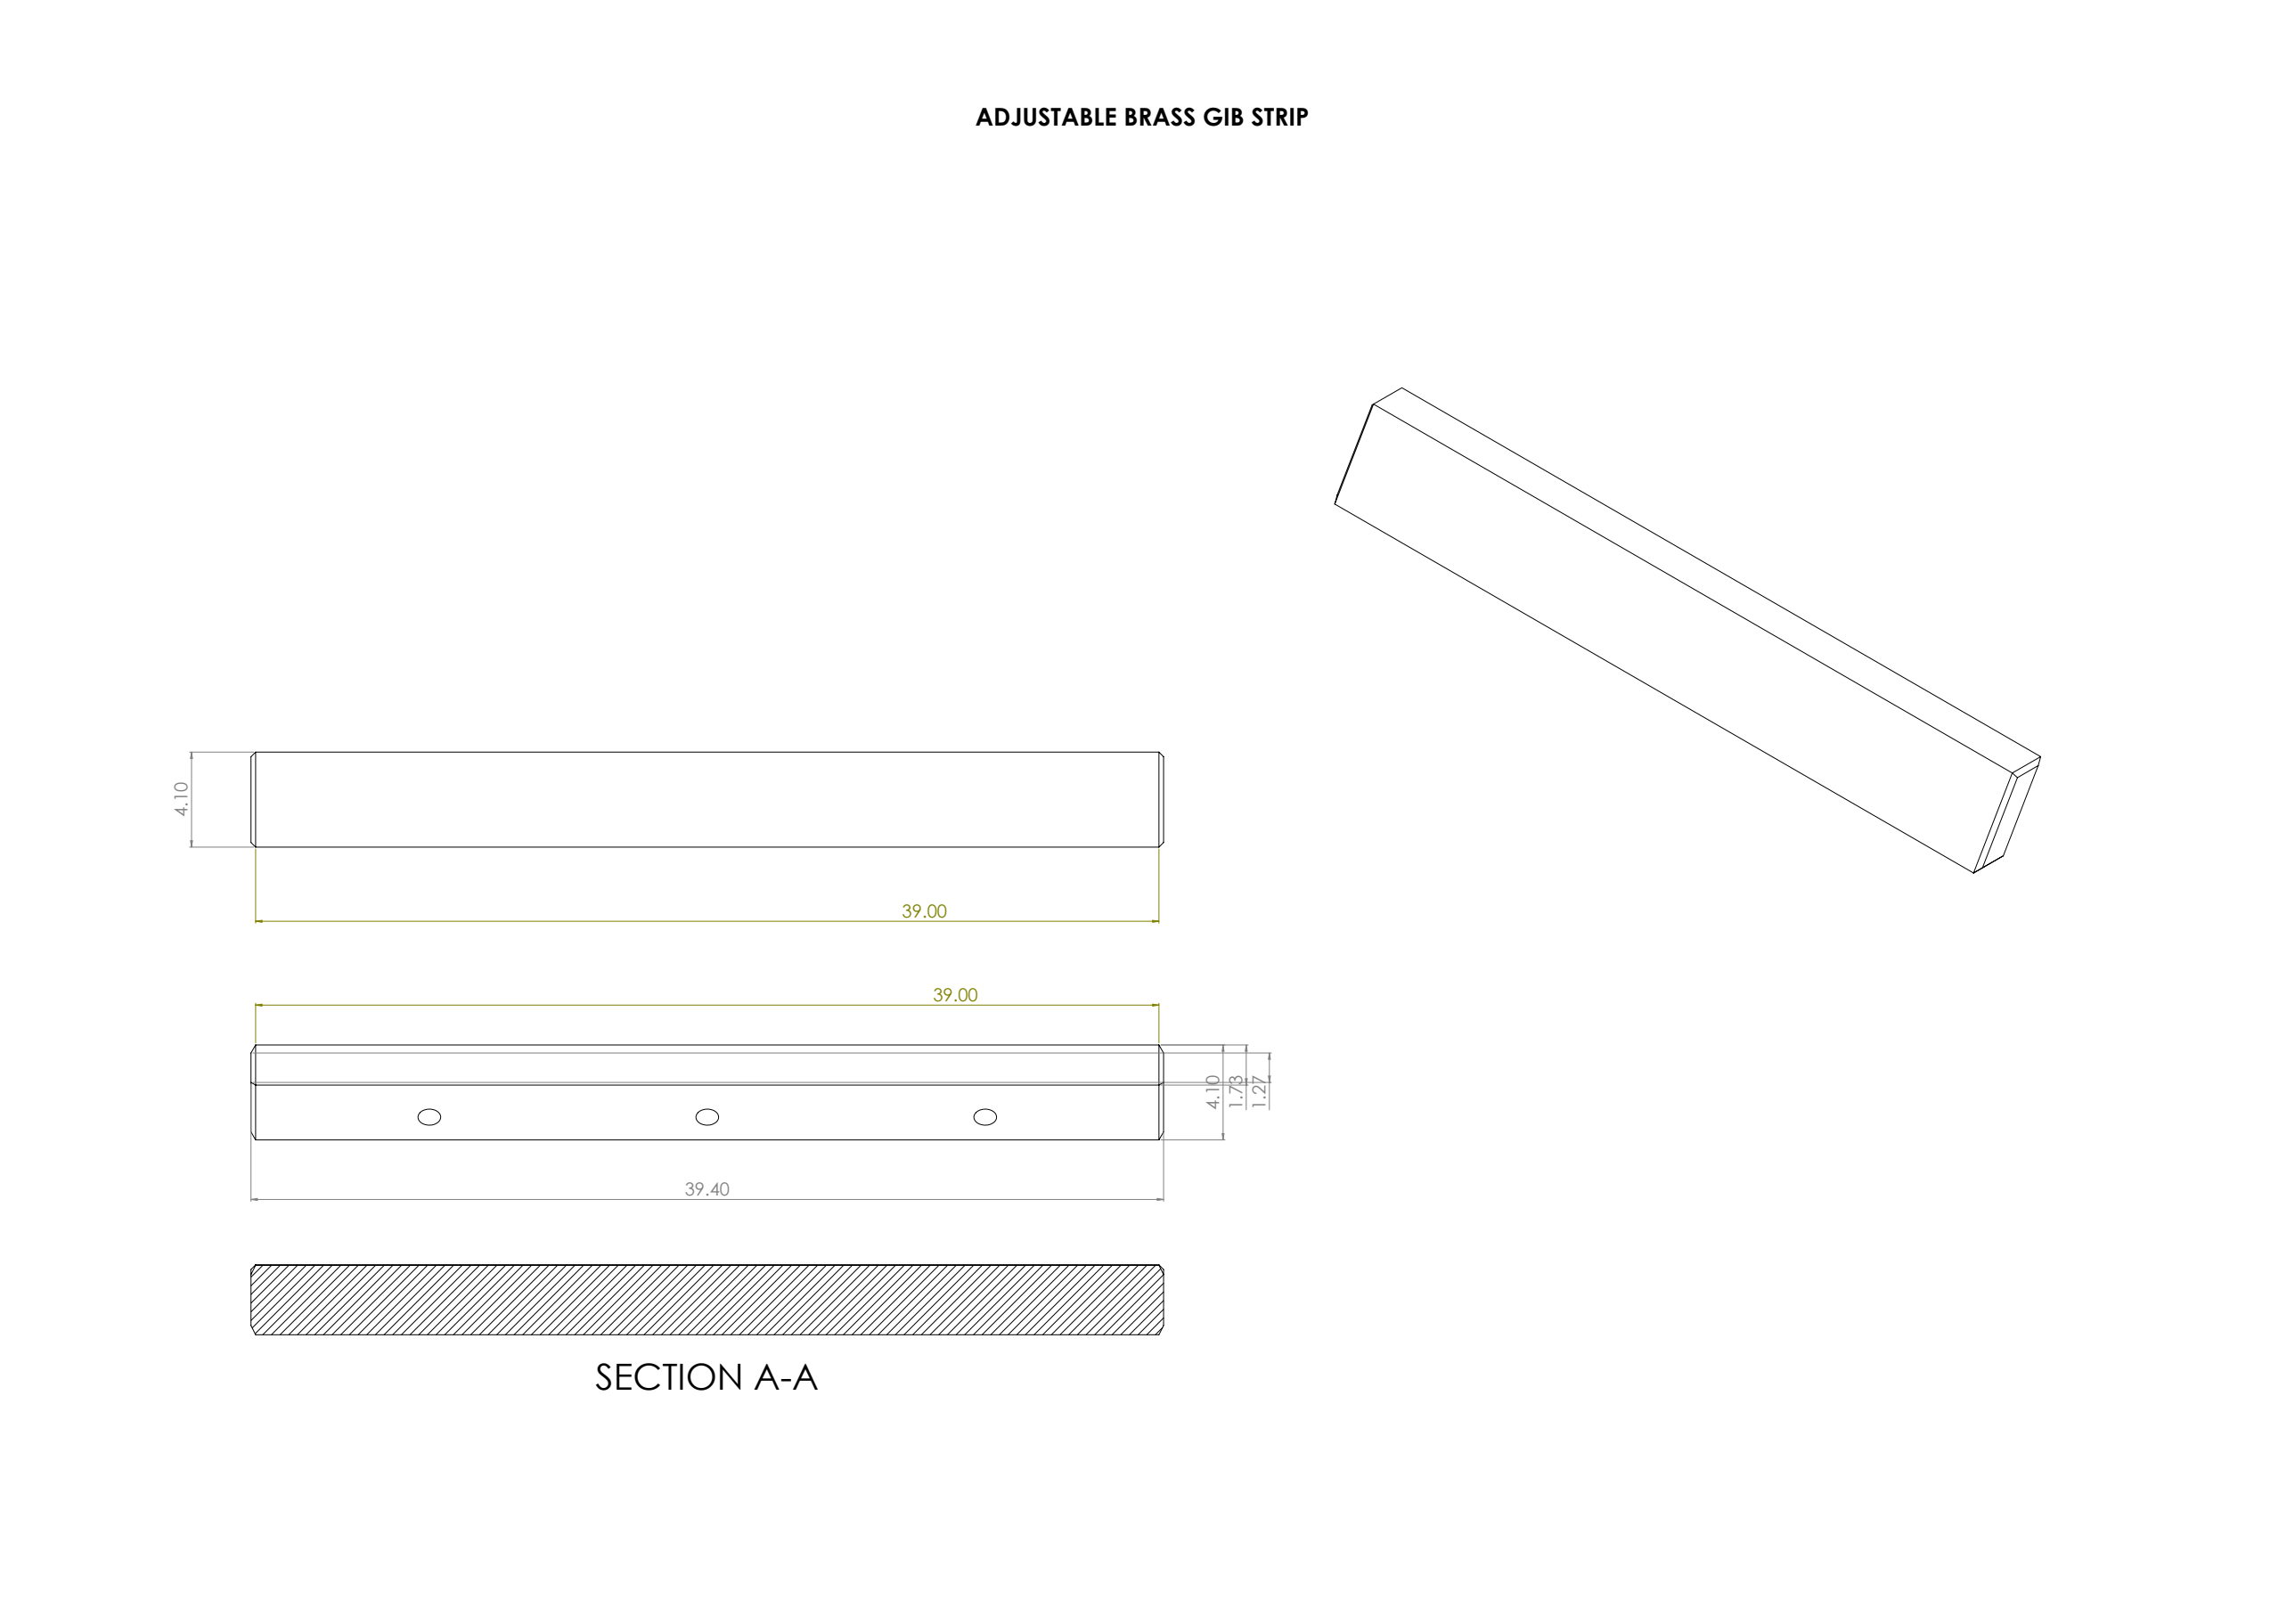
ISO-10303-21;
HEADER;
/* Generated by software containing ST-Developer
 * from STEP Tools, Inc. (www.steptools.com) 
 */

FILE_DESCRIPTION(
/* description */ (''),
/* implementation_level */ '2;1');

FILE_NAME(
/* name */ 'Adjustable Brass Gib Strip.step',
/* time_stamp */ '2026-10-05T09:57:53+05:00',
/* author */ (''),
/* organization */ (''),
/* preprocessor_version */ 'ST-DEVELOPER v20.2',
/* originating_system */ 'Autodesk Translation Framework v15.15.0.0',
/* authorisation */ '');

FILE_SCHEMA (('AUTOMOTIVE_DESIGN { 1 0 10303 214 3 1 1 }'));
ENDSEC;

DATA;
#10=MECHANICAL_DESIGN_GEOMETRIC_PRESENTATION_REPRESENTATION('',(#553),#113984);
#517=SHAPE_REPRESENTATION_RELATIONSHIP('SRR','None',#114054,#535);
#535=ADVANCED_BREP_SHAPE_REPRESENTATION('',(#571),#113968);
#553=STYLED_ITEM('',(#114324),#571);
#571=MANIFOLD_SOLID_BREP('Adjustable Brass Gib Strip',#60394);
#598=ELLIPSE('',#61950,0.692820323027559,0.489897948556646);
#599=ELLIPSE('',#61952,0.692820323027559,0.489897948556646);
#600=ELLIPSE('',#61954,0.692820323027559,0.489897948556646);
#908=CONICAL_SURFACE('',#61949,1.40000000000001,0.78539816339745);
#909=CONICAL_SURFACE('',#61951,1.40000000000001,0.78539816339745);
#910=CONICAL_SURFACE('',#61953,1.40000000000001,0.78539816339745);
#1822=FACE_BOUND('',#9512,.T.);
#1823=FACE_BOUND('',#9513,.T.);
#1824=FACE_BOUND('',#9514,.T.);
#3021=PLANE('',#61955);
#3022=PLANE('',#61956);
#3023=PLANE('',#61957);
#3024=PLANE('',#61958);
#3025=PLANE('',#61959);
#3026=PLANE('',#61960);
#3027=PLANE('',#61961);
#3028=PLANE('',#61962);
#3029=PLANE('',#61963);
#3030=PLANE('',#61964);
#3031=PLANE('',#61965);
#3032=PLANE('',#61966);
#3033=PLANE('',#61967);
#3034=PLANE('',#61968);
#5950=FACE_OUTER_BOUND('',#9497,.T.);
#5951=FACE_OUTER_BOUND('',#9498,.T.);
#5952=FACE_OUTER_BOUND('',#9499,.T.);
#5953=FACE_OUTER_BOUND('',#9500,.T.);
#5954=FACE_OUTER_BOUND('',#9501,.T.);
#5955=FACE_OUTER_BOUND('',#9502,.T.);
#5956=FACE_OUTER_BOUND('',#9503,.T.);
#5957=FACE_OUTER_BOUND('',#9504,.T.);
#5958=FACE_OUTER_BOUND('',#9505,.T.);
#5959=FACE_OUTER_BOUND('',#9506,.T.);
#5960=FACE_OUTER_BOUND('',#9507,.T.);
#5961=FACE_OUTER_BOUND('',#9508,.T.);
#5962=FACE_OUTER_BOUND('',#9509,.T.);
#5963=FACE_OUTER_BOUND('',#9510,.T.);
#5964=FACE_OUTER_BOUND('',#9511,.T.);
#5965=FACE_OUTER_BOUND('',#9515,.T.);
#5966=FACE_OUTER_BOUND('',#9516,.T.);
#9497=EDGE_LOOP('',(#48881,#48882,#48883));
#9498=EDGE_LOOP('',(#48884,#48885,#48886));
#9499=EDGE_LOOP('',(#48887,#48888,#48889));
#9500=EDGE_LOOP('',(#48890,#48891,#48892,#48893));
#9501=EDGE_LOOP('',(#48894,#48895,#48896,#48897));
#9502=EDGE_LOOP('',(#48898,#48899,#48900,#48901));
#9503=EDGE_LOOP('',(#48902,#48903,#48904,#48905));
#9504=EDGE_LOOP('',(#48906,#48907,#48908,#48909));
#9505=EDGE_LOOP('',(#48910,#48911,#48912,#48913));
#9506=EDGE_LOOP('',(#48914,#48915,#48916,#48917));
#9507=EDGE_LOOP('',(#48918,#48919,#48920,#48921));
#9508=EDGE_LOOP('',(#48922,#48923,#48924,#48925));
#9509=EDGE_LOOP('',(#48926,#48927,#48928,#48929));
#9510=EDGE_LOOP('',(#48930,#48931,#48932,#48933));
#9511=EDGE_LOOP('',(#48934,#48935,#48936,#48937));
#9512=EDGE_LOOP('',(#48938));
#9513=EDGE_LOOP('',(#48939));
#9514=EDGE_LOOP('',(#48940));
#9515=EDGE_LOOP('',(#48941,#48942,#48943,#48944));
#9516=EDGE_LOOP('',(#48945,#48946,#48947,#48948));
#14287=LINE('',#92544,#20321);
#14288=LINE('',#92549,#20322);
#14289=LINE('',#92554,#20323);
#14290=LINE('',#92558,#20324);
#14291=LINE('',#92560,#20325);
#14292=LINE('',#92562,#20326);
#14293=LINE('',#92563,#20327);
#14294=LINE('',#92566,#20328);
#14295=LINE('',#92568,#20329);
#14296=LINE('',#92569,#20330);
#14297=LINE('',#92572,#20331);
#14298=LINE('',#92574,#20332);
#14299=LINE('',#92575,#20333);
#14300=LINE('',#92577,#20334);
#14301=LINE('',#92578,#20335);
#14302=LINE('',#92581,#20336);
#14303=LINE('',#92583,#20337);
#14304=LINE('',#92584,#20338);
#14305=LINE('',#92587,#20339);
#14306=LINE('',#92588,#20340);
#14307=LINE('',#92593,#20341);
#14308=LINE('',#92594,#20342);
#14309=LINE('',#92595,#20343);
#14310=LINE('',#92598,#20344);
#14311=LINE('',#92599,#20345);
#14312=LINE('',#92602,#20346);
#14313=LINE('',#92604,#20347);
#14314=LINE('',#92605,#20348);
#14315=LINE('',#92607,#20349);
#14316=LINE('',#92608,#20350);
#14317=LINE('',#92610,#20351);
#20321=VECTOR('',#69871,1.40000000000001);
#20322=VECTOR('',#69876,1.40000000000001);
#20323=VECTOR('',#69881,1.40000000000001);
#20324=VECTOR('',#69884,10.);
#20325=VECTOR('',#69885,10.);
#20326=VECTOR('',#69886,10.);
#20327=VECTOR('',#69887,10.);
#20328=VECTOR('',#69890,10.);
#20329=VECTOR('',#69891,10.);
#20330=VECTOR('',#69892,10.);
#20331=VECTOR('',#69895,10.);
#20332=VECTOR('',#69896,10.);
#20333=VECTOR('',#69897,10.);
#20334=VECTOR('',#69900,10.);
#20335=VECTOR('',#69901,10.);
#20336=VECTOR('',#69904,10.);
#20337=VECTOR('',#69905,10.);
#20338=VECTOR('',#69906,10.);
#20339=VECTOR('',#69909,10.);
#20340=VECTOR('',#69910,10.);
#20341=VECTOR('',#69915,10.);
#20342=VECTOR('',#69916,10.);
#20343=VECTOR('',#69917,10.);
#20344=VECTOR('',#69920,10.);
#20345=VECTOR('',#69921,10.);
#20346=VECTOR('',#69924,10.);
#20347=VECTOR('',#69925,10.);
#20348=VECTOR('',#69926,10.);
#20349=VECTOR('',#69929,10.);
#20350=VECTOR('',#69930,10.);
#20351=VECTOR('',#69933,10.);
#27877=VERTEX_POINT('',#92541);
#27878=VERTEX_POINT('',#92543);
#27879=VERTEX_POINT('',#92546);
#27880=VERTEX_POINT('',#92548);
#27881=VERTEX_POINT('',#92551);
#27882=VERTEX_POINT('',#92553);
#27883=VERTEX_POINT('',#92556);
#27884=VERTEX_POINT('',#92557);
#27885=VERTEX_POINT('',#92559);
#27886=VERTEX_POINT('',#92561);
#27887=VERTEX_POINT('',#92565);
#27888=VERTEX_POINT('',#92567);
#27889=VERTEX_POINT('',#92571);
#27890=VERTEX_POINT('',#92573);
#27891=VERTEX_POINT('',#92580);
#27892=VERTEX_POINT('',#92582);
#27893=VERTEX_POINT('',#92586);
#27894=VERTEX_POINT('',#92591);
#27895=VERTEX_POINT('',#92592);
#27896=VERTEX_POINT('',#92597);
#27897=VERTEX_POINT('',#92601);
#27898=VERTEX_POINT('',#92603);
#35273=EDGE_CURVE('',#27877,#27877,#598,.T.);
#35274=EDGE_CURVE('',#27877,#27878,#14287,.T.);
#35275=EDGE_CURVE('',#27879,#27879,#599,.T.);
#35276=EDGE_CURVE('',#27879,#27880,#14288,.T.);
#35277=EDGE_CURVE('',#27881,#27881,#600,.T.);
#35278=EDGE_CURVE('',#27881,#27882,#14289,.T.);
#35279=EDGE_CURVE('',#27883,#27884,#14290,.T.);
#35280=EDGE_CURVE('',#27884,#27885,#14291,.T.);
#35281=EDGE_CURVE('',#27885,#27886,#14292,.T.);
#35282=EDGE_CURVE('',#27883,#27886,#14293,.T.);
#35283=EDGE_CURVE('',#27884,#27887,#14294,.T.);
#35284=EDGE_CURVE('',#27887,#27888,#14295,.T.);
#35285=EDGE_CURVE('',#27888,#27885,#14296,.T.);
#35286=EDGE_CURVE('',#27887,#27889,#14297,.T.);
#35287=EDGE_CURVE('',#27889,#27890,#14298,.T.);
#35288=EDGE_CURVE('',#27890,#27888,#14299,.T.);
#35289=EDGE_CURVE('',#27886,#27890,#14300,.T.);
#35290=EDGE_CURVE('',#27889,#27883,#14301,.T.);
#35291=EDGE_CURVE('',#27891,#27886,#14302,.T.);
#35292=EDGE_CURVE('',#27892,#27891,#14303,.T.);
#35293=EDGE_CURVE('',#27892,#27890,#14304,.T.);
#35294=EDGE_CURVE('',#27893,#27885,#14305,.T.);
#35295=EDGE_CURVE('',#27891,#27893,#14306,.T.);
#35296=EDGE_CURVE('',#27894,#27895,#14307,.T.);
#35297=EDGE_CURVE('',#27895,#27891,#14308,.T.);
#35298=EDGE_CURVE('',#27894,#27893,#14309,.T.);
#35299=EDGE_CURVE('',#27895,#27896,#14310,.T.);
#35300=EDGE_CURVE('',#27896,#27892,#14311,.T.);
#35301=EDGE_CURVE('',#27893,#27897,#14312,.T.);
#35302=EDGE_CURVE('',#27897,#27898,#14313,.T.);
#35303=EDGE_CURVE('',#27898,#27894,#14314,.T.);
#35304=EDGE_CURVE('',#27896,#27898,#14315,.T.);
#35305=EDGE_CURVE('',#27897,#27892,#14316,.T.);
#35306=EDGE_CURVE('',#27897,#27888,#14317,.T.);
#48881=ORIENTED_EDGE('',*,*,#35273,.F.);
#48882=ORIENTED_EDGE('',*,*,#35274,.T.);
#48883=ORIENTED_EDGE('',*,*,#35274,.F.);
#48884=ORIENTED_EDGE('',*,*,#35275,.F.);
#48885=ORIENTED_EDGE('',*,*,#35276,.T.);
#48886=ORIENTED_EDGE('',*,*,#35276,.F.);
#48887=ORIENTED_EDGE('',*,*,#35277,.F.);
#48888=ORIENTED_EDGE('',*,*,#35278,.T.);
#48889=ORIENTED_EDGE('',*,*,#35278,.F.);
#48890=ORIENTED_EDGE('',*,*,#35279,.T.);
#48891=ORIENTED_EDGE('',*,*,#35280,.T.);
#48892=ORIENTED_EDGE('',*,*,#35281,.T.);
#48893=ORIENTED_EDGE('',*,*,#35282,.F.);
#48894=ORIENTED_EDGE('',*,*,#35283,.T.);
#48895=ORIENTED_EDGE('',*,*,#35284,.T.);
#48896=ORIENTED_EDGE('',*,*,#35285,.T.);
#48897=ORIENTED_EDGE('',*,*,#35280,.F.);
#48898=ORIENTED_EDGE('',*,*,#35286,.T.);
#48899=ORIENTED_EDGE('',*,*,#35287,.T.);
#48900=ORIENTED_EDGE('',*,*,#35288,.T.);
#48901=ORIENTED_EDGE('',*,*,#35284,.F.);
#48902=ORIENTED_EDGE('',*,*,#35289,.T.);
#48903=ORIENTED_EDGE('',*,*,#35287,.F.);
#48904=ORIENTED_EDGE('',*,*,#35290,.T.);
#48905=ORIENTED_EDGE('',*,*,#35282,.T.);
#48906=ORIENTED_EDGE('',*,*,#35289,.F.);
#48907=ORIENTED_EDGE('',*,*,#35291,.F.);
#48908=ORIENTED_EDGE('',*,*,#35292,.F.);
#48909=ORIENTED_EDGE('',*,*,#35293,.T.);
#48910=ORIENTED_EDGE('',*,*,#35281,.F.);
#48911=ORIENTED_EDGE('',*,*,#35294,.F.);
#48912=ORIENTED_EDGE('',*,*,#35295,.F.);
#48913=ORIENTED_EDGE('',*,*,#35291,.T.);
#48914=ORIENTED_EDGE('',*,*,#35279,.F.);
#48915=ORIENTED_EDGE('',*,*,#35290,.F.);
#48916=ORIENTED_EDGE('',*,*,#35286,.F.);
#48917=ORIENTED_EDGE('',*,*,#35283,.F.);
#48918=ORIENTED_EDGE('',*,*,#35296,.T.);
#48919=ORIENTED_EDGE('',*,*,#35297,.T.);
#48920=ORIENTED_EDGE('',*,*,#35295,.T.);
#48921=ORIENTED_EDGE('',*,*,#35298,.F.);
#48922=ORIENTED_EDGE('',*,*,#35299,.T.);
#48923=ORIENTED_EDGE('',*,*,#35300,.T.);
#48924=ORIENTED_EDGE('',*,*,#35292,.T.);
#48925=ORIENTED_EDGE('',*,*,#35297,.F.);
#48926=ORIENTED_EDGE('',*,*,#35301,.T.);
#48927=ORIENTED_EDGE('',*,*,#35302,.T.);
#48928=ORIENTED_EDGE('',*,*,#35303,.T.);
#48929=ORIENTED_EDGE('',*,*,#35298,.T.);
#48930=ORIENTED_EDGE('',*,*,#35304,.T.);
#48931=ORIENTED_EDGE('',*,*,#35302,.F.);
#48932=ORIENTED_EDGE('',*,*,#35305,.T.);
#48933=ORIENTED_EDGE('',*,*,#35300,.F.);
#48934=ORIENTED_EDGE('',*,*,#35285,.F.);
#48935=ORIENTED_EDGE('',*,*,#35306,.F.);
#48936=ORIENTED_EDGE('',*,*,#35301,.F.);
#48937=ORIENTED_EDGE('',*,*,#35294,.T.);
#48938=ORIENTED_EDGE('',*,*,#35273,.T.);
#48939=ORIENTED_EDGE('',*,*,#35275,.T.);
#48940=ORIENTED_EDGE('',*,*,#35277,.T.);
#48941=ORIENTED_EDGE('',*,*,#35296,.F.);
#48942=ORIENTED_EDGE('',*,*,#35303,.F.);
#48943=ORIENTED_EDGE('',*,*,#35304,.F.);
#48944=ORIENTED_EDGE('',*,*,#35299,.F.);
#48945=ORIENTED_EDGE('',*,*,#35288,.F.);
#48946=ORIENTED_EDGE('',*,*,#35293,.F.);
#48947=ORIENTED_EDGE('',*,*,#35305,.F.);
#48948=ORIENTED_EDGE('',*,*,#35306,.T.);
#59050=ADVANCED_FACE('',(#5950),#908,.F.);
#59051=ADVANCED_FACE('',(#5951),#909,.F.);
#59052=ADVANCED_FACE('',(#5952),#910,.F.);
#59053=ADVANCED_FACE('',(#5953),#3021,.T.);
#59054=ADVANCED_FACE('',(#5954),#3022,.T.);
#59055=ADVANCED_FACE('',(#5955),#3023,.T.);
#59056=ADVANCED_FACE('',(#5956),#3024,.T.);
#59057=ADVANCED_FACE('',(#5957),#3025,.T.);
#59058=ADVANCED_FACE('',(#5958),#3026,.T.);
#59059=ADVANCED_FACE('',(#5959),#3027,.T.);
#59060=ADVANCED_FACE('',(#5960),#3028,.T.);
#59061=ADVANCED_FACE('',(#5961),#3029,.T.);
#59062=ADVANCED_FACE('',(#5962),#3030,.T.);
#59063=ADVANCED_FACE('',(#5963),#3031,.T.);
#59064=ADVANCED_FACE('',(#5964,#1822,#1823,#1824),#3032,.T.);
#59065=ADVANCED_FACE('',(#5965),#3033,.F.);
#59066=ADVANCED_FACE('',(#5966),#3034,.T.);
#60394=CLOSED_SHELL('',(#59050,#59051,#59052,#59053,#59054,#59055,#59056,
#59057,#59058,#59059,#59060,#59061,#59062,#59063,#59064,#59065,#59066));
#61948=AXIS2_PLACEMENT_3D('',#92539,#69865,#69866);
#61949=AXIS2_PLACEMENT_3D('',#92540,#69867,#69868);
#61950=AXIS2_PLACEMENT_3D('',#92542,#69869,#69870);
#61951=AXIS2_PLACEMENT_3D('',#92545,#69872,#69873);
#61952=AXIS2_PLACEMENT_3D('',#92547,#69874,#69875);
#61953=AXIS2_PLACEMENT_3D('',#92550,#69877,#69878);
#61954=AXIS2_PLACEMENT_3D('',#92552,#69879,#69880);
#61955=AXIS2_PLACEMENT_3D('',#92555,#69882,#69883);
#61956=AXIS2_PLACEMENT_3D('',#92564,#69888,#69889);
#61957=AXIS2_PLACEMENT_3D('',#92570,#69893,#69894);
#61958=AXIS2_PLACEMENT_3D('',#92576,#69898,#69899);
#61959=AXIS2_PLACEMENT_3D('',#92579,#69902,#69903);
#61960=AXIS2_PLACEMENT_3D('',#92585,#69907,#69908);
#61961=AXIS2_PLACEMENT_3D('',#92589,#69911,#69912);
#61962=AXIS2_PLACEMENT_3D('',#92590,#69913,#69914);
#61963=AXIS2_PLACEMENT_3D('',#92596,#69918,#69919);
#61964=AXIS2_PLACEMENT_3D('',#92600,#69922,#69923);
#61965=AXIS2_PLACEMENT_3D('',#92606,#69927,#69928);
#61966=AXIS2_PLACEMENT_3D('',#92609,#69931,#69932);
#61967=AXIS2_PLACEMENT_3D('',#92611,#69934,#69935);
#61968=AXIS2_PLACEMENT_3D('',#92612,#69936,#69937);
#69865=DIRECTION('axis',(0.,0.,1.));
#69866=DIRECTION('refdir',(1.,0.,0.));
#69867=DIRECTION('center_axis',(0.,0.,-1.));
#69868=DIRECTION('ref_axis',(1.,0.,0.));
#69869=DIRECTION('center_axis',(0.,0.5,0.866025403784439));
#69870=DIRECTION('ref_axis',(2.56395024851139E-14,-0.866025403784439,0.5));
#69871=DIRECTION('',(0.707106781186549,8.65956056235495E-17,0.707106781186546));
#69872=DIRECTION('center_axis',(0.,0.,-1.));
#69873=DIRECTION('ref_axis',(1.,0.,0.));
#69874=DIRECTION('center_axis',(0.,0.5,0.866025403784439));
#69875=DIRECTION('ref_axis',(2.56395024851139E-14,-0.866025403784439,0.5));
#69876=DIRECTION('',(0.707106781186549,8.65956056235495E-17,0.707106781186546));
#69877=DIRECTION('center_axis',(0.,0.,-1.));
#69878=DIRECTION('ref_axis',(1.,0.,0.));
#69879=DIRECTION('center_axis',(0.,0.5,0.866025403784439));
#69880=DIRECTION('ref_axis',(2.56395024851139E-14,-0.866025403784439,0.5));
#69881=DIRECTION('',(0.707106781186549,8.65956056235495E-17,0.707106781186546));
#69882=DIRECTION('center_axis',(0.707106781186555,0.70710678118654,0.));
#69883=DIRECTION('ref_axis',(0.,0.,-1.));
#69884=DIRECTION('',(0.,0.,-1.));
#69885=DIRECTION('',(-0.447213595499949,0.447213595499959,-0.774596669241488));
#69886=DIRECTION('',(0.,0.,1.));
#69887=DIRECTION('',(-0.654653670707967,0.654653670707982,0.377964473009236));
#69888=DIRECTION('center_axis',(0.707106781186556,-0.35355339059327,-0.612372435695787));
#69889=DIRECTION('ref_axis',(-0.654653670707968,0.,-0.755928946018463));
#69890=DIRECTION('',(0.,-0.866025403784439,0.5));
#69891=DIRECTION('',(-0.654653670707969,-0.654653670707984,-0.37796447300923));
#69892=DIRECTION('',(0.,0.866025403784439,-0.5));
#69893=DIRECTION('center_axis',(0.707106781186555,-0.70710678118654,0.));
#69894=DIRECTION('ref_axis',(0.,0.,-1.));
#69895=DIRECTION('',(0.,0.,1.));
#69896=DIRECTION('',(-0.447213595499949,-0.447213595499959,0.774596669241488));
#69897=DIRECTION('',(0.,0.,-1.));
#69898=DIRECTION('center_axis',(0.707106781186556,0.35355339059327,0.612372435695787));
#69899=DIRECTION('ref_axis',(0.654653670707968,0.,-0.755928946018463));
#69900=DIRECTION('',(0.,-0.866025403784439,0.5));
#69901=DIRECTION('',(0.,0.866025403784439,-0.5));
#69902=DIRECTION('center_axis',(0.,0.5,0.866025403784439));
#69903=DIRECTION('ref_axis',(0.,-0.866025403784439,0.5));
#69904=DIRECTION('',(1.,0.,0.));
#69905=DIRECTION('',(0.,0.866025403784439,-0.5));
#69906=DIRECTION('',(1.,0.,0.));
#69907=DIRECTION('center_axis',(0.,1.,0.));
#69908=DIRECTION('ref_axis',(0.,0.,1.));
#69909=DIRECTION('',(1.,0.,0.));
#69910=DIRECTION('',(0.,0.,-1.));
#69911=DIRECTION('center_axis',(1.,0.,0.));
#69912=DIRECTION('ref_axis',(0.,0.,-1.));
#69913=DIRECTION('center_axis',(-0.707106781186555,0.70710678118654,0.));
#69914=DIRECTION('ref_axis',(0.,0.,1.));
#69915=DIRECTION('',(0.,0.,1.));
#69916=DIRECTION('',(0.654653670707967,0.654653670707982,0.377964473009236));
#69917=DIRECTION('',(0.447213595499949,0.447213595499959,-0.774596669241488));
#69918=DIRECTION('center_axis',(-0.707106781186556,0.35355339059327,0.612372435695787));
#69919=DIRECTION('ref_axis',(0.654653670707968,0.,0.755928946018463));
#69920=DIRECTION('',(0.,-0.866025403784439,0.5));
#69921=DIRECTION('',(0.447213595499949,-0.447213595499959,0.774596669241488));
#69922=DIRECTION('center_axis',(-0.707106781186556,-0.35355339059327,-0.612372435695787));
#69923=DIRECTION('ref_axis',(-0.654653670707968,0.,0.755928946018463));
#69924=DIRECTION('',(0.,-0.866025403784439,0.5));
#69925=DIRECTION('',(-0.654653670707969,0.654653670707984,0.37796447300923));
#69926=DIRECTION('',(0.,0.866025403784439,-0.5));
#69927=DIRECTION('center_axis',(-0.707106781186555,-0.70710678118654,0.));
#69928=DIRECTION('ref_axis',(0.,0.,1.));
#69929=DIRECTION('',(0.,0.,-1.));
#69930=DIRECTION('',(0.,0.,1.));
#69931=DIRECTION('center_axis',(0.,-0.5,-0.866025403784439));
#69932=DIRECTION('ref_axis',(0.,0.866025403784439,-0.5));
#69933=DIRECTION('',(1.,0.,0.));
#69934=DIRECTION('center_axis',(1.,0.,0.));
#69935=DIRECTION('ref_axis',(0.,0.,-1.));
#69936=DIRECTION('center_axis',(0.,-1.,0.));
#69937=DIRECTION('ref_axis',(0.,0.,-1.));
#92539=CARTESIAN_POINT('',(0.,0.,0.));
#92540=CARTESIAN_POINT('Origin',(110.,10.75,14.5323462819564));
#92541=CARTESIAN_POINT('',(109.6,10.75,15.5323462819564));
#92542=CARTESIAN_POINT('Origin',(110.,11.0964101615138,15.3323462819564));
#92543=CARTESIAN_POINT('',(110.,10.75,15.9323462819564));
#92544=CARTESIAN_POINT('',(108.6,10.75,14.5323462819564));
#92545=CARTESIAN_POINT('Origin',(122.,10.75,14.5323462819564));
#92546=CARTESIAN_POINT('',(121.6,10.75,15.5323462819564));
#92547=CARTESIAN_POINT('Origin',(122.,11.0964101615138,15.3323462819564));
#92548=CARTESIAN_POINT('',(122.,10.75,15.9323462819564));
#92549=CARTESIAN_POINT('',(120.6,10.75,14.5323462819564));
#92550=CARTESIAN_POINT('Origin',(98.,10.75,14.5323462819564));
#92551=CARTESIAN_POINT('',(97.6,10.75,15.5323462819564));
#92552=CARTESIAN_POINT('Origin',(98.,11.0964101615138,15.3323462819564));
#92553=CARTESIAN_POINT('',(98.,10.75,15.9323462819564));
#92554=CARTESIAN_POINT('',(96.6,10.75,14.5323462819564));
#92555=CARTESIAN_POINT('Origin',(129.6,12.7,15.3735749579293));
#92556=CARTESIAN_POINT('',(129.7,12.6,15.9653589838486));
#92557=CARTESIAN_POINT('',(129.7,12.6,14.6951883916314));
#92558=CARTESIAN_POINT('',(129.7,12.6,15.3735749579293));
#92559=CARTESIAN_POINT('',(129.5,12.8,14.3487782301177));
#92560=CARTESIAN_POINT('',(129.7,12.6,14.6951883916314));
#92561=CARTESIAN_POINT('',(129.5,12.8,16.0808290376865));
#92562=CARTESIAN_POINT('',(129.5,12.8,15.3735749579293));
#92563=CARTESIAN_POINT('',(129.7,12.6,15.9653589838486));
#92564=CARTESIAN_POINT('Origin',(129.6,9.5875,16.3189860237273));
#92565=CARTESIAN_POINT('',(129.7,8.9,16.8313843876331));
#92566=CARTESIAN_POINT('',(129.7,9.6375,16.4055885641057));
#92567=CARTESIAN_POINT('',(129.5,8.7,16.7159143337951));
#92568=CARTESIAN_POINT('',(129.7,8.9,16.8313843876331));
#92569=CARTESIAN_POINT('',(129.5,9.5375,16.2323834833488));
#92570=CARTESIAN_POINT('Origin',(129.6,8.8,17.4231684135524));
#92571=CARTESIAN_POINT('',(129.7,8.9,18.1015549798502));
#92572=CARTESIAN_POINT('',(129.7,8.9,17.4231684135524));
#92573=CARTESIAN_POINT('',(129.5,8.7,18.447965141364));
#92574=CARTESIAN_POINT('',(129.7,8.9,18.1015549798502));
#92575=CARTESIAN_POINT('',(129.5,8.7,17.4231684135524));
#92576=CARTESIAN_POINT('Origin',(129.6,11.9125,16.4777573477544));
#92577=CARTESIAN_POINT('',(129.5,11.9625,16.5643598881329));
#92578=CARTESIAN_POINT('',(129.7,11.8625,16.391154807376));
#92579=CARTESIAN_POINT('Origin',(90.3,12.8,16.0808290376865));
#92580=CARTESIAN_POINT('',(90.5,12.8,16.0808290376865));
#92581=CARTESIAN_POINT('',(90.3,12.8,16.0808290376865));
#92582=CARTESIAN_POINT('',(90.5,8.7,18.447965141364));
#92583=CARTESIAN_POINT('',(90.5,11.9625,16.5643598881329));
#92584=CARTESIAN_POINT('',(90.3,8.7,18.447965141364));
#92585=CARTESIAN_POINT('Origin',(90.3,12.8,14.3487782301177));
#92586=CARTESIAN_POINT('',(90.5,12.8,14.3487782301177));
#92587=CARTESIAN_POINT('',(90.3,12.8,14.3487782301177));
#92588=CARTESIAN_POINT('',(90.5,12.8,15.3735749579293));
#92589=CARTESIAN_POINT('Origin',(129.7,10.75,16.3983716857408));
#92590=CARTESIAN_POINT('Origin',(90.4,12.7,15.3735749579293));
#92591=CARTESIAN_POINT('',(90.3,12.6,14.6951883916314));
#92592=CARTESIAN_POINT('',(90.3,12.6,15.9653589838486));
#92593=CARTESIAN_POINT('',(90.3,12.6,15.3735749579293));
#92594=CARTESIAN_POINT('',(90.3,12.6,15.9653589838486));
#92595=CARTESIAN_POINT('',(90.3,12.6,14.6951883916314));
#92596=CARTESIAN_POINT('Origin',(90.4,11.9125,16.4777573477544));
#92597=CARTESIAN_POINT('',(90.3,8.9,18.1015549798502));
#92598=CARTESIAN_POINT('',(90.3,11.8625,16.391154807376));
#92599=CARTESIAN_POINT('',(90.3,8.9,18.1015549798502));
#92600=CARTESIAN_POINT('Origin',(90.4,9.5875,16.3189860237273));
#92601=CARTESIAN_POINT('',(90.5,8.7,16.7159143337951));
#92602=CARTESIAN_POINT('',(90.5,9.5375,16.2323834833488));
#92603=CARTESIAN_POINT('',(90.3,8.9,16.8313843876331));
#92604=CARTESIAN_POINT('',(90.5,8.7,16.7159143337951));
#92605=CARTESIAN_POINT('',(90.3,9.6375,16.4055885641057));
#92606=CARTESIAN_POINT('Origin',(90.4,8.8,17.4231684135524));
#92607=CARTESIAN_POINT('',(90.3,8.9,17.4231684135524));
#92608=CARTESIAN_POINT('',(90.5,8.7,17.4231684135524));
#92609=CARTESIAN_POINT('Origin',(90.3,8.7,16.7159143337951));
#92610=CARTESIAN_POINT('',(90.3,8.7,16.7159143337951));
#92611=CARTESIAN_POINT('Origin',(90.3,10.75,16.3983716857408));
#92612=CARTESIAN_POINT('Origin',(90.3,8.7,18.447965141364));
#113948=UNCERTAINTY_MEASURE_WITH_UNIT(LENGTH_MEASURE(0.01),#113985,
'DISTANCE_ACCURACY_VALUE',
'Maximum model space distance between geometric entities at asserted c
onnectivities');
#113964=UNCERTAINTY_MEASURE_WITH_UNIT(LENGTH_MEASURE(0.01),#113985,
'DISTANCE_ACCURACY_VALUE',
'Maximum model space distance between geometric entities at asserted c
onnectivities');
#113968=(
GEOMETRIC_REPRESENTATION_CONTEXT(3)
GLOBAL_UNCERTAINTY_ASSIGNED_CONTEXT((#113948))
GLOBAL_UNIT_ASSIGNED_CONTEXT((#113985,#113987,#113988))
REPRESENTATION_CONTEXT('','3D')
);
#113984=(
GEOMETRIC_REPRESENTATION_CONTEXT(3)
GLOBAL_UNCERTAINTY_ASSIGNED_CONTEXT((#113964))
GLOBAL_UNIT_ASSIGNED_CONTEXT((#113985,#113987,#113988))
REPRESENTATION_CONTEXT('','3D')
);
#113985=(
LENGTH_UNIT()
NAMED_UNIT(*)
SI_UNIT(.MILLI.,.METRE.)
);
#113987=(
NAMED_UNIT(*)
PLANE_ANGLE_UNIT()
SI_UNIT($,.RADIAN.)
);
#113988=(
NAMED_UNIT(*)
SI_UNIT($,.STERADIAN.)
SOLID_ANGLE_UNIT()
);
#113992=SHAPE_DEFINITION_REPRESENTATION(#114011,#114054);
#114011=PRODUCT_DEFINITION_SHAPE('',$,#114074);
#114054=SHAPE_REPRESENTATION('',(#61948),#113968);
#114070=PRODUCT_DEFINITION_CONTEXT('part definition',#114129,'design');
#114074=PRODUCT_DEFINITION('2026-10-05-09-48-59-239',
'Adjustable Brass Gib Strip',#114093,#114070);
#114093=PRODUCT_DEFINITION_FORMATION('',$,#114134);
#114129=APPLICATION_CONTEXT(
'Core Data for Automotive Mechanical Design Process');
#114130=PRODUCT_CONTEXT('part definition',#114129,'mechanical');
#114134=PRODUCT('2026-10-05-09-48-59-239','Adjustable Brass Gib Strip',
$,(#114130));
#114318=COLOUR_RGB('Off White',0.89,0.88,0.83);
#114319=FILL_AREA_STYLE_COLOUR('',#114318);
#114320=FILL_AREA_STYLE('',(#114319));
#114321=SURFACE_STYLE_FILL_AREA(#114320);
#114322=SURFACE_SIDE_STYLE('',(#114321));
#114323=SURFACE_STYLE_USAGE(.BOTH.,#114322);
#114324=PRESENTATION_STYLE_ASSIGNMENT((#114323));
ENDSEC;
END-ISO-10303-21;
